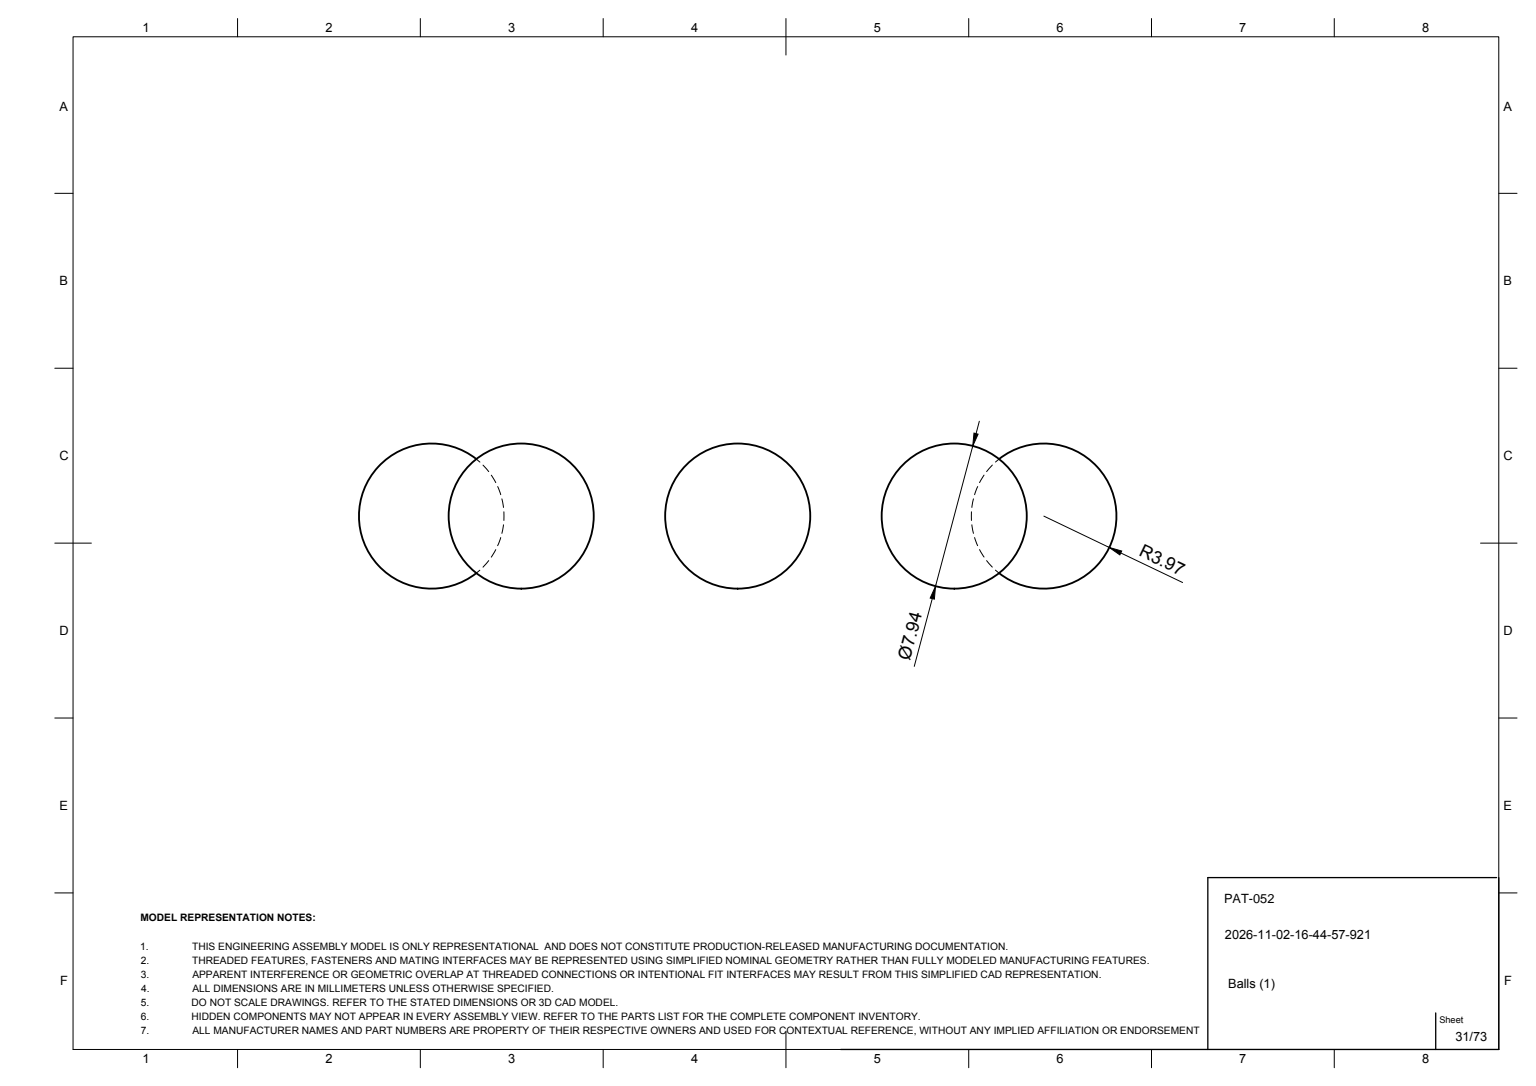
ISO-10303-21;
HEADER;
/* Generated by software containing ST-Developer
 * from STEP Tools, Inc. (www.steptools.com) 
 */

FILE_DESCRIPTION(
/* description */ ('Hand-crank gear train demonstrator'),
/* implementation_level */ '2;1');

FILE_NAME(
/* name */ 'Balls (1).step',
/* time_stamp */ '2026-10-28T03:22:13-07:00',
/* author */ (''),
/* organization */ (''),
/* preprocessor_version */ 'ST-DEVELOPER v20.2',
/* originating_system */ 'Autodesk Translation Framework v15.17.0.0',
/* authorisation */ '');

FILE_SCHEMA (('AUTOMOTIVE_DESIGN { 1 0 10303 214 3 1 1 }'));
ENDSEC;

DATA;
#10=MECHANICAL_DESIGN_GEOMETRIC_PRESENTATION_REPRESENTATION('',(#1214,#1215,#1216,#1217,#1218,#1219,#1220,#1221),#62758);
#1005=SPHERICAL_SURFACE('',#17654,0.3969);
#1006=SPHERICAL_SURFACE('',#17656,0.3969);
#1007=SPHERICAL_SURFACE('',#17658,0.3969);
#1008=SPHERICAL_SURFACE('',#17660,0.3969);
#1009=SPHERICAL_SURFACE('',#17662,0.3969);
#1010=SPHERICAL_SURFACE('',#17664,0.3969);
#1011=SPHERICAL_SURFACE('',#17666,0.3969);
#1012=SPHERICAL_SURFACE('',#17668,0.3969);
#1079=SHAPE_REPRESENTATION_RELATIONSHIP('SRR','None',#63053,#1143);
#1143=ADVANCED_BREP_SHAPE_REPRESENTATION('',(#1292,#1293,#1294,#1295,#1296,
#1297,#1298,#1299),#62707);
#1214=STYLED_ITEM('',(#63462),#1292);
#1215=STYLED_ITEM('',(#63462),#1293);
#1216=STYLED_ITEM('',(#63462),#1294);
#1217=STYLED_ITEM('',(#63462),#1295);
#1218=STYLED_ITEM('',(#63462),#1296);
#1219=STYLED_ITEM('',(#63462),#1297);
#1220=STYLED_ITEM('',(#63462),#1298);
#1221=STYLED_ITEM('',(#63462),#1299);
#1292=MANIFOLD_SOLID_BREP('Body1',#16395);
#1293=MANIFOLD_SOLID_BREP('Body2',#16396);
#1294=MANIFOLD_SOLID_BREP('Body3',#16397);
#1295=MANIFOLD_SOLID_BREP('Body4',#16398);
#1296=MANIFOLD_SOLID_BREP('Body5',#16399);
#1297=MANIFOLD_SOLID_BREP('Body6',#16400);
#1298=MANIFOLD_SOLID_BREP('Body7',#16401);
#1299=MANIFOLD_SOLID_BREP('Body8',#16402);
#2325=FACE_OUTER_BOUND('',#3419,.T.);
#2326=FACE_OUTER_BOUND('',#3420,.T.);
#2327=FACE_OUTER_BOUND('',#3421,.T.);
#2328=FACE_OUTER_BOUND('',#3422,.T.);
#2329=FACE_OUTER_BOUND('',#3423,.T.);
#2330=FACE_OUTER_BOUND('',#3424,.T.);
#2331=FACE_OUTER_BOUND('',#3425,.T.);
#2332=FACE_OUTER_BOUND('',#3426,.T.);
#3419=EDGE_LOOP('',(#11721,#11722));
#3420=EDGE_LOOP('',(#11723,#11724));
#3421=EDGE_LOOP('',(#11725,#11726));
#3422=EDGE_LOOP('',(#11727,#11728));
#3423=EDGE_LOOP('',(#11729,#11730));
#3424=EDGE_LOOP('',(#11731,#11732));
#3425=EDGE_LOOP('',(#11733,#11734));
#3426=EDGE_LOOP('',(#11735,#11736));
#6816=CIRCLE('',#17655,0.3969);
#6817=CIRCLE('',#17657,0.3969);
#6818=CIRCLE('',#17659,0.3969);
#6819=CIRCLE('',#17661,0.3969);
#6820=CIRCLE('',#17663,0.3969);
#6821=CIRCLE('',#17665,0.3969);
#6822=CIRCLE('',#17667,0.3969);
#6823=CIRCLE('',#17669,0.3969);
#7513=VERTEX_POINT('',#24578);
#7514=VERTEX_POINT('',#24579);
#7515=VERTEX_POINT('',#24582);
#7516=VERTEX_POINT('',#24583);
#7517=VERTEX_POINT('',#24586);
#7518=VERTEX_POINT('',#24587);
#7519=VERTEX_POINT('',#24590);
#7520=VERTEX_POINT('',#24591);
#7521=VERTEX_POINT('',#24594);
#7522=VERTEX_POINT('',#24595);
#7523=VERTEX_POINT('',#24598);
#7524=VERTEX_POINT('',#24599);
#7525=VERTEX_POINT('',#24602);
#7526=VERTEX_POINT('',#24603);
#7527=VERTEX_POINT('',#24606);
#7528=VERTEX_POINT('',#24607);
#9112=EDGE_CURVE('',#7513,#7514,#6816,.T.);
#9113=EDGE_CURVE('',#7515,#7516,#6817,.T.);
#9114=EDGE_CURVE('',#7517,#7518,#6818,.T.);
#9115=EDGE_CURVE('',#7519,#7520,#6819,.T.);
#9116=EDGE_CURVE('',#7521,#7522,#6820,.T.);
#9117=EDGE_CURVE('',#7523,#7524,#6821,.T.);
#9118=EDGE_CURVE('',#7525,#7526,#6822,.T.);
#9119=EDGE_CURVE('',#7527,#7528,#6823,.T.);
#11721=ORIENTED_EDGE('',*,*,#9112,.T.);
#11722=ORIENTED_EDGE('',*,*,#9112,.F.);
#11723=ORIENTED_EDGE('',*,*,#9113,.T.);
#11724=ORIENTED_EDGE('',*,*,#9113,.F.);
#11725=ORIENTED_EDGE('',*,*,#9114,.T.);
#11726=ORIENTED_EDGE('',*,*,#9114,.F.);
#11727=ORIENTED_EDGE('',*,*,#9115,.T.);
#11728=ORIENTED_EDGE('',*,*,#9115,.F.);
#11729=ORIENTED_EDGE('',*,*,#9116,.T.);
#11730=ORIENTED_EDGE('',*,*,#9116,.F.);
#11731=ORIENTED_EDGE('',*,*,#9117,.T.);
#11732=ORIENTED_EDGE('',*,*,#9117,.F.);
#11733=ORIENTED_EDGE('',*,*,#9118,.T.);
#11734=ORIENTED_EDGE('',*,*,#9118,.F.);
#11735=ORIENTED_EDGE('',*,*,#9119,.T.);
#11736=ORIENTED_EDGE('',*,*,#9119,.F.);
#15635=ADVANCED_FACE('',(#2325),#1005,.T.);
#15636=ADVANCED_FACE('',(#2326),#1006,.T.);
#15637=ADVANCED_FACE('',(#2327),#1007,.T.);
#15638=ADVANCED_FACE('',(#2328),#1008,.T.);
#15639=ADVANCED_FACE('',(#2329),#1009,.T.);
#15640=ADVANCED_FACE('',(#2330),#1010,.T.);
#15641=ADVANCED_FACE('',(#2331),#1011,.T.);
#15642=ADVANCED_FACE('',(#2332),#1012,.T.);
#16395=CLOSED_SHELL('',(#15635));
#16396=CLOSED_SHELL('',(#15636));
#16397=CLOSED_SHELL('',(#15637));
#16398=CLOSED_SHELL('',(#15638));
#16399=CLOSED_SHELL('',(#15639));
#16400=CLOSED_SHELL('',(#15640));
#16401=CLOSED_SHELL('',(#15641));
#16402=CLOSED_SHELL('',(#15642));
#17653=AXIS2_PLACEMENT_3D('',#24576,#19984,#19985);
#17654=AXIS2_PLACEMENT_3D('',#24577,#19986,#19987);
#17655=AXIS2_PLACEMENT_3D('',#24580,#19988,#19989);
#17656=AXIS2_PLACEMENT_3D('',#24581,#19990,#19991);
#17657=AXIS2_PLACEMENT_3D('',#24584,#19992,#19993);
#17658=AXIS2_PLACEMENT_3D('',#24585,#19994,#19995);
#17659=AXIS2_PLACEMENT_3D('',#24588,#19996,#19997);
#17660=AXIS2_PLACEMENT_3D('',#24589,#19998,#19999);
#17661=AXIS2_PLACEMENT_3D('',#24592,#20000,#20001);
#17662=AXIS2_PLACEMENT_3D('',#24593,#20002,#20003);
#17663=AXIS2_PLACEMENT_3D('',#24596,#20004,#20005);
#17664=AXIS2_PLACEMENT_3D('',#24597,#20006,#20007);
#17665=AXIS2_PLACEMENT_3D('',#24600,#20008,#20009);
#17666=AXIS2_PLACEMENT_3D('',#24601,#20010,#20011);
#17667=AXIS2_PLACEMENT_3D('',#24604,#20012,#20013);
#17668=AXIS2_PLACEMENT_3D('',#24605,#20014,#20015);
#17669=AXIS2_PLACEMENT_3D('',#24608,#20016,#20017);
#19984=DIRECTION('axis',(0.,0.,1.));
#19985=DIRECTION('refdir',(1.,0.,0.));
#19986=DIRECTION('center_axis',(0.,0.,1.));
#19987=DIRECTION('ref_axis',(1.,0.,0.));
#19988=DIRECTION('center_axis',(1.22464679914735E-16,-1.,0.));
#19989=DIRECTION('ref_axis',(-1.,-1.22464679914735E-16,0.));
#19990=DIRECTION('center_axis',(0.707106781186548,0.,0.707106781186548));
#19991=DIRECTION('ref_axis',(0.707106781186548,0.,-0.707106781186548));
#19992=DIRECTION('center_axis',(8.65956056235493E-17,-1.,-8.65956056235493E-17));
#19993=DIRECTION('ref_axis',(-0.707106781186548,-1.22464679914735E-16,0.707106781186548));
#19994=DIRECTION('center_axis',(1.,0.,0.));
#19995=DIRECTION('ref_axis',(6.12323399573677E-17,0.,-1.));
#19996=DIRECTION('center_axis',(7.49879891330929E-33,-1.,-1.22464679914735E-16));
#19997=DIRECTION('ref_axis',(-6.12323399573677E-17,-1.22464679914735E-16,
1.));
#19998=DIRECTION('center_axis',(0.707106781186548,0.,-0.707106781186548));
#19999=DIRECTION('ref_axis',(-0.707106781186548,0.,-0.707106781186548));
#20000=DIRECTION('center_axis',(-8.65956056235493E-17,-1.,-8.65956056235493E-17));
#20001=DIRECTION('ref_axis',(0.707106781186548,-1.22464679914735E-16,0.707106781186548));
#20002=DIRECTION('center_axis',(0.,0.,-1.));
#20003=DIRECTION('ref_axis',(-1.,0.,-1.22464679914735E-16));
#20004=DIRECTION('center_axis',(-1.22464679914735E-16,-1.,-1.49975978266186E-32));
#20005=DIRECTION('ref_axis',(1.,-1.22464679914735E-16,1.22464679914735E-16));
#20006=DIRECTION('center_axis',(-0.707106781186548,0.,-0.707106781186548));
#20007=DIRECTION('ref_axis',(-0.707106781186548,0.,0.707106781186548));
#20008=DIRECTION('center_axis',(-8.65956056235493E-17,-1.,8.65956056235493E-17));
#20009=DIRECTION('ref_axis',(0.707106781186548,-1.22464679914735E-16,-0.707106781186548));
#20010=DIRECTION('center_axis',(-1.,0.,0.));
#20011=DIRECTION('ref_axis',(-1.83697019872103E-16,0.,1.));
#20012=DIRECTION('center_axis',(-2.24963967399279E-32,-1.,1.22464679914735E-16));
#20013=DIRECTION('ref_axis',(1.83697019872103E-16,-1.22464679914735E-16,
-1.));
#20014=DIRECTION('center_axis',(-0.707106781186548,0.,0.707106781186548));
#20015=DIRECTION('ref_axis',(0.707106781186548,0.,0.707106781186548));
#20016=DIRECTION('center_axis',(8.65956056235493E-17,-1.,8.65956056235494E-17));
#20017=DIRECTION('ref_axis',(-0.707106781186548,-1.22464679914735E-16,-0.707106781186548));
#24576=CARTESIAN_POINT('',(0.,0.,0.));
#24577=CARTESIAN_POINT('Origin',(1.675,0.,0.));
#24578=CARTESIAN_POINT('',(1.675,-2.97627328869245E-33,0.3969));
#24579=CARTESIAN_POINT('',(1.675,-2.97627328869245E-33,-0.3969));
#24580=CARTESIAN_POINT('Origin',(1.675,0.,0.));
#24581=CARTESIAN_POINT('Origin',(1.18440385848747,0.,-1.18440385848747));
#24582=CARTESIAN_POINT('',(1.46505453994041,3.1867025333467E-33,-0.903753177034526));
#24583=CARTESIAN_POINT('',(0.903753177034527,-9.13924911073161E-33,-1.46505453994041));
#24584=CARTESIAN_POINT('Origin',(1.18440385848747,0.,-1.18440385848747));
#24585=CARTESIAN_POINT('Origin',(1.02564169428591E-16,0.,-1.675));
#24586=CARTESIAN_POINT('',(0.3969,-2.97627328869246E-33,-1.675));
#24587=CARTESIAN_POINT('',(-0.3969,-2.97627328869245E-33,-1.675));
#24588=CARTESIAN_POINT('Origin',(1.02564169428591E-16,0.,-1.675));
#24589=CARTESIAN_POINT('Origin',(-1.18440385848747,0.,-1.18440385848747));
#24590=CARTESIAN_POINT('',(-0.903753177034526,3.1867025333467E-33,-1.46505453994041));
#24591=CARTESIAN_POINT('',(-1.46505453994041,-9.13924911073161E-33,-0.903753177034527));
#24592=CARTESIAN_POINT('Origin',(-1.18440385848747,0.,-1.18440385848747));
#24593=CARTESIAN_POINT('Origin',(-1.675,0.,-2.05128338857182E-16));
#24594=CARTESIAN_POINT('',(-1.675,-2.97627328869246E-33,-0.3969));
#24595=CARTESIAN_POINT('',(-1.675,-2.97627328869245E-33,0.3969));
#24596=CARTESIAN_POINT('Origin',(-1.675,0.,-2.05128338857182E-16));
#24597=CARTESIAN_POINT('Origin',(-1.18440385848747,0.,1.18440385848747));
#24598=CARTESIAN_POINT('',(-1.46505453994041,6.26819044436628E-33,0.903753177034526));
#24599=CARTESIAN_POINT('',(-0.903753177034527,-1.22207370217512E-32,1.46505453994041));
#24600=CARTESIAN_POINT('Origin',(-1.18440385848747,0.,1.18440385848747));
#24601=CARTESIAN_POINT('Origin',(-3.07692508285772E-16,0.,1.675));
#24602=CARTESIAN_POINT('',(-0.3969,-2.97627328869246E-33,1.675));
#24603=CARTESIAN_POINT('',(0.396899999999999,-2.97627328869245E-33,1.675));
#24604=CARTESIAN_POINT('Origin',(-3.07692508285772E-16,0.,1.675));
#24605=CARTESIAN_POINT('Origin',(1.18440385848747,0.,1.18440385848747));
#24606=CARTESIAN_POINT('',(0.903753177034526,9.34967835538585E-33,1.46505453994041));
#24607=CARTESIAN_POINT('',(1.46505453994041,-1.53022249327708E-32,0.903753177034527));
#24608=CARTESIAN_POINT('Origin',(1.18440385848747,0.,1.18440385848747));
#62633=UNCERTAINTY_MEASURE_WITH_UNIT(LENGTH_MEASURE(0.001),#62759,
'DISTANCE_ACCURACY_VALUE',
'Maximum model space distance between geometric entities at asserted c
onnectivities');
#62684=UNCERTAINTY_MEASURE_WITH_UNIT(LENGTH_MEASURE(0.001),#62759,
'DISTANCE_ACCURACY_VALUE',
'Maximum model space distance between geometric entities at asserted c
onnectivities');
#62707=(
GEOMETRIC_REPRESENTATION_CONTEXT(3)
GLOBAL_UNCERTAINTY_ASSIGNED_CONTEXT((#62633))
GLOBAL_UNIT_ASSIGNED_CONTEXT((#62759,#62761,#62762))
REPRESENTATION_CONTEXT('','3D')
);
#62758=(
GEOMETRIC_REPRESENTATION_CONTEXT(3)
GLOBAL_UNCERTAINTY_ASSIGNED_CONTEXT((#62684))
GLOBAL_UNIT_ASSIGNED_CONTEXT((#62759,#62761,#62762))
REPRESENTATION_CONTEXT('','3D')
);
#62759=(
LENGTH_UNIT()
NAMED_UNIT(*)
SI_UNIT(.CENTI.,.METRE.)
);
#62761=(
NAMED_UNIT(*)
PLANE_ANGLE_UNIT()
SI_UNIT($,.RADIAN.)
);
#62762=(
NAMED_UNIT(*)
SI_UNIT($,.STERADIAN.)
SOLID_ANGLE_UNIT()
);
#62785=SHAPE_DEFINITION_REPRESENTATION(#62863,#63053);
#62863=PRODUCT_DEFINITION_SHAPE('',$,#63127);
#63053=SHAPE_REPRESENTATION('',(#17653),#62707);
#63104=PRODUCT_DEFINITION_CONTEXT('part definition',#63325,'design');
#63127=PRODUCT_DEFINITION('Balls (1)','Balls (1)',#63200,#63104);
#63200=PRODUCT_DEFINITION_FORMATION('',$,#63349);
#63325=APPLICATION_CONTEXT(
'Core Data for Automotive Mechanical Design Process');
#63326=PRODUCT_CONTEXT('part definition',#63325,'mechanical');
#63349=PRODUCT('Balls (1)','Balls (1)','Balls (1)',(#63326));
#63456=COLOUR_RGB('Grey',0.48,0.52,0.57);
#63457=FILL_AREA_STYLE_COLOUR('',#63456);
#63458=FILL_AREA_STYLE('',(#63457));
#63459=SURFACE_STYLE_FILL_AREA(#63458);
#63460=SURFACE_SIDE_STYLE('',(#63459));
#63461=SURFACE_STYLE_USAGE(.BOTH.,#63460);
#63462=PRESENTATION_STYLE_ASSIGNMENT((#63461));
ENDSEC;
END-ISO-10303-21;
